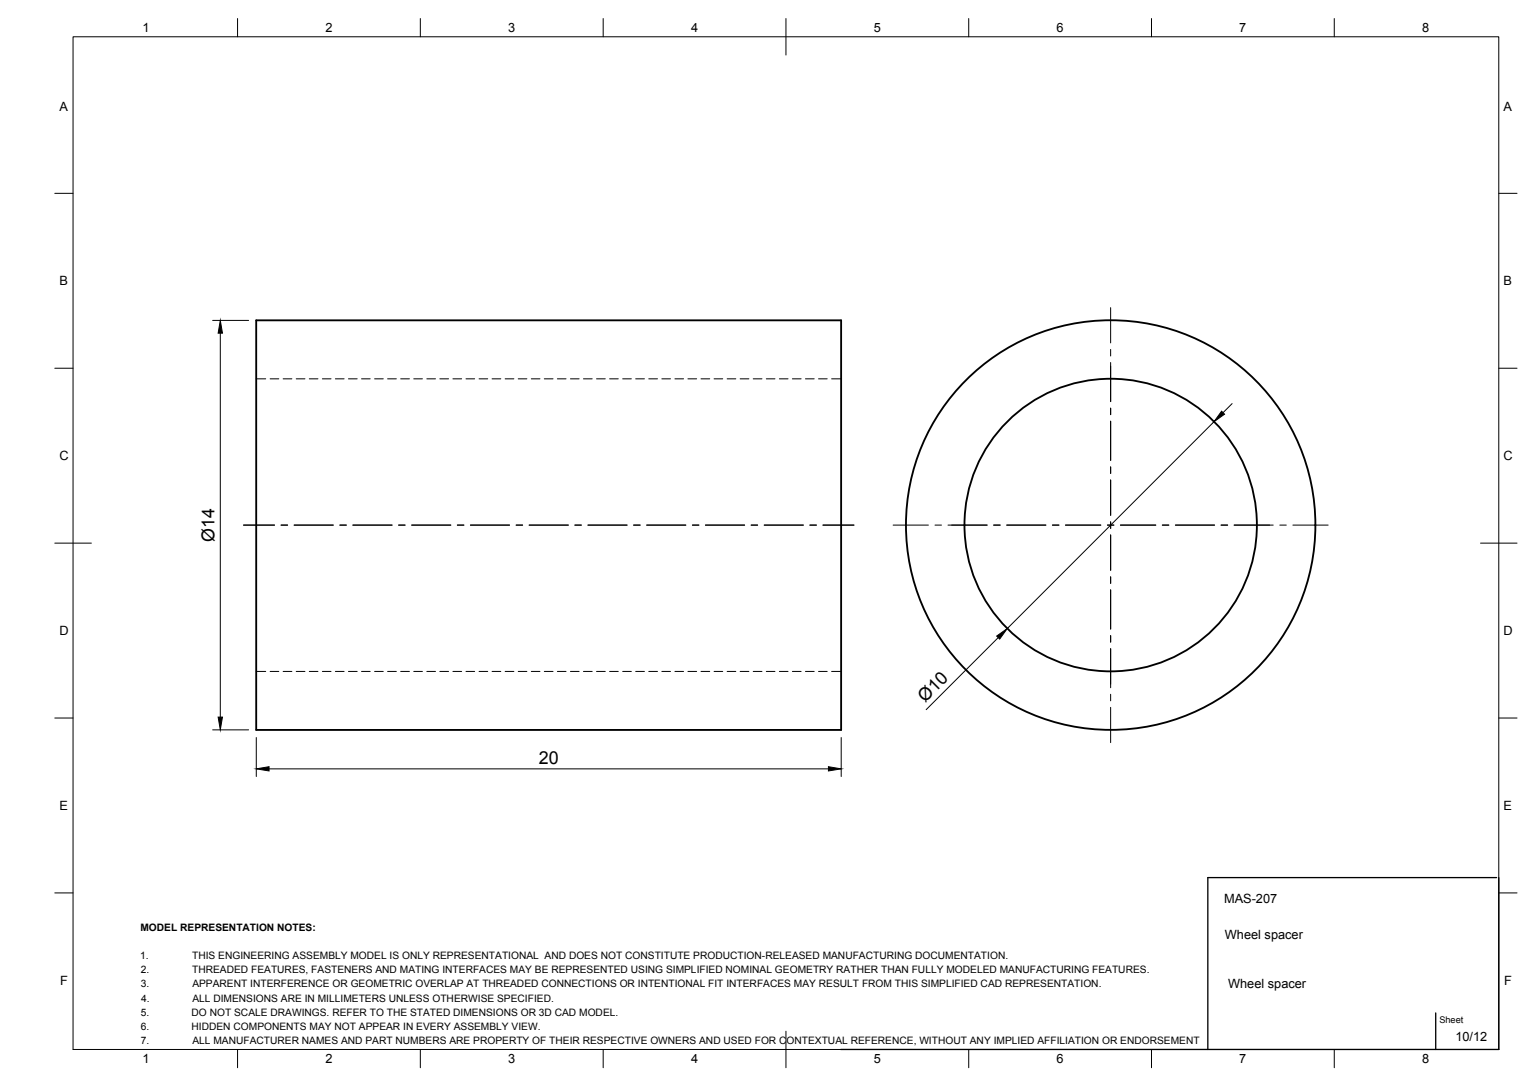
ISO-10303-21;
HEADER;
/* Generated by software containing ST-Developer
 * from STEP Tools, Inc. (www.steptools.com) 
 */

FILE_DESCRIPTION(
/* description */ ('Independent six-slot Geneva indexer. Center distance100, drive radius
50, 60degree indexing per input revolution with120degree engagement an
d240degree dwell. Native machined concave locking faces and relieved d
isk; replaceable retained drive pin; keyed output shaft. Geometry traj
ectory checks use calculated indexing positions, not a contact-dynamic
s simulation. No load or production rating assigned.'),
/* implementation_level */ '2;1');

FILE_NAME(
/* name */ 'Wheel spacer.step',
/* time_stamp */ '2026-11-09T17:53:22-08:00',
/* author */ (''),
/* organization */ (''),
/* preprocessor_version */ 'ST-DEVELOPER v20.2',
/* originating_system */ 'Autodesk Translation Framework v15.17.0.0',
/* authorisation */ '');

FILE_SCHEMA (('AUTOMOTIVE_DESIGN { 1 0 10303 214 3 1 1 }'));
ENDSEC;

DATA;
#10=MECHANICAL_DESIGN_GEOMETRIC_PRESENTATION_REPRESENTATION('',(#108),#4149);
#86=SHAPE_REPRESENTATION_RELATIONSHIP('SRR','None',#4203,#97);
#97=ADVANCED_BREP_SHAPE_REPRESENTATION('',(#119),#4145);
#108=STYLED_ITEM('',(#4266),#119);
#119=MANIFOLD_SOLID_BREP('Body1',#2302);
#155=FACE_BOUND('',#527,.T.);
#156=FACE_BOUND('',#529,.T.);
#228=PLANE('',#2669);
#229=PLANE('',#2670);
#356=FACE_OUTER_BOUND('',#524,.T.);
#357=FACE_OUTER_BOUND('',#525,.T.);
#358=FACE_OUTER_BOUND('',#526,.T.);
#359=FACE_OUTER_BOUND('',#528,.T.);
#524=EDGE_LOOP('',(#2040,#2041,#2042,#2043));
#525=EDGE_LOOP('',(#2044,#2045,#2046,#2047));
#526=EDGE_LOOP('',(#2048));
#527=EDGE_LOOP('',(#2049));
#528=EDGE_LOOP('',(#2050));
#529=EDGE_LOOP('',(#2051));
#706=LINE('',#4040,#878);
#707=LINE('',#4046,#879);
#878=VECTOR('',#3349,5.);
#879=VECTOR('',#3356,7.);
#1000=CIRCLE('',#2664,5.);
#1001=CIRCLE('',#2665,5.);
#1002=CIRCLE('',#2667,7.);
#1003=CIRCLE('',#2668,7.);
#1192=VERTEX_POINT('',#4037);
#1193=VERTEX_POINT('',#4039);
#1194=VERTEX_POINT('',#4043);
#1195=VERTEX_POINT('',#4045);
#1478=EDGE_CURVE('',#1192,#1192,#1000,.T.);
#1479=EDGE_CURVE('',#1192,#1193,#706,.T.);
#1480=EDGE_CURVE('',#1193,#1193,#1001,.T.);
#1481=EDGE_CURVE('',#1194,#1194,#1002,.T.);
#1482=EDGE_CURVE('',#1194,#1195,#707,.T.);
#1483=EDGE_CURVE('',#1195,#1195,#1003,.T.);
#2040=ORIENTED_EDGE('',*,*,#1478,.F.);
#2041=ORIENTED_EDGE('',*,*,#1479,.T.);
#2042=ORIENTED_EDGE('',*,*,#1480,.T.);
#2043=ORIENTED_EDGE('',*,*,#1479,.F.);
#2044=ORIENTED_EDGE('',*,*,#1481,.F.);
#2045=ORIENTED_EDGE('',*,*,#1482,.T.);
#2046=ORIENTED_EDGE('',*,*,#1483,.T.);
#2047=ORIENTED_EDGE('',*,*,#1482,.F.);
#2048=ORIENTED_EDGE('',*,*,#1481,.T.);
#2049=ORIENTED_EDGE('',*,*,#1478,.T.);
#2050=ORIENTED_EDGE('',*,*,#1483,.F.);
#2051=ORIENTED_EDGE('',*,*,#1480,.F.);
#2151=CYLINDRICAL_SURFACE('',#2663,5.);
#2152=CYLINDRICAL_SURFACE('',#2666,7.);
#2277=ADVANCED_FACE('',(#356),#2151,.F.);
#2278=ADVANCED_FACE('',(#357),#2152,.T.);
#2279=ADVANCED_FACE('',(#358,#155),#228,.T.);
#2280=ADVANCED_FACE('',(#359,#156),#229,.F.);
#2302=CLOSED_SHELL('',(#2277,#2278,#2279,#2280));
#2662=AXIS2_PLACEMENT_3D('',#4035,#3343,#3344);
#2663=AXIS2_PLACEMENT_3D('',#4036,#3345,#3346);
#2664=AXIS2_PLACEMENT_3D('',#4038,#3347,#3348);
#2665=AXIS2_PLACEMENT_3D('',#4041,#3350,#3351);
#2666=AXIS2_PLACEMENT_3D('',#4042,#3352,#3353);
#2667=AXIS2_PLACEMENT_3D('',#4044,#3354,#3355);
#2668=AXIS2_PLACEMENT_3D('',#4047,#3357,#3358);
#2669=AXIS2_PLACEMENT_3D('',#4048,#3359,#3360);
#2670=AXIS2_PLACEMENT_3D('',#4049,#3361,#3362);
#3343=DIRECTION('axis',(0.,0.,1.));
#3344=DIRECTION('refdir',(1.,0.,0.));
#3345=DIRECTION('center_axis',(0.,0.,1.));
#3346=DIRECTION('ref_axis',(1.,0.,0.));
#3347=DIRECTION('center_axis',(0.,0.,-1.));
#3348=DIRECTION('ref_axis',(1.,0.,0.));
#3349=DIRECTION('',(0.,0.,-1.));
#3350=DIRECTION('center_axis',(0.,0.,-1.));
#3351=DIRECTION('ref_axis',(1.,0.,0.));
#3352=DIRECTION('center_axis',(0.,0.,1.));
#3353=DIRECTION('ref_axis',(1.,0.,0.));
#3354=DIRECTION('center_axis',(0.,0.,1.));
#3355=DIRECTION('ref_axis',(1.,0.,0.));
#3356=DIRECTION('',(0.,0.,-1.));
#3357=DIRECTION('center_axis',(0.,0.,1.));
#3358=DIRECTION('ref_axis',(1.,0.,0.));
#3359=DIRECTION('center_axis',(0.,0.,1.));
#3360=DIRECTION('ref_axis',(1.,0.,0.));
#3361=DIRECTION('center_axis',(0.,0.,1.));
#3362=DIRECTION('ref_axis',(1.,0.,0.));
#4035=CARTESIAN_POINT('',(0.,0.,0.));
#4036=CARTESIAN_POINT('Origin',(0.,0.,0.));
#4037=CARTESIAN_POINT('',(-5.,-6.12323399573677E-16,20.));
#4038=CARTESIAN_POINT('Origin',(0.,0.,20.));
#4039=CARTESIAN_POINT('',(-5.,-6.12323399573677E-16,0.));
#4040=CARTESIAN_POINT('',(-5.,-6.12323399573677E-16,0.));
#4041=CARTESIAN_POINT('Origin',(0.,0.,0.));
#4042=CARTESIAN_POINT('Origin',(0.,0.,0.));
#4043=CARTESIAN_POINT('',(-7.,-8.57252759403147E-16,20.));
#4044=CARTESIAN_POINT('Origin',(0.,0.,20.));
#4045=CARTESIAN_POINT('',(-7.,-8.57252759403147E-16,0.));
#4046=CARTESIAN_POINT('',(-7.,-8.57252759403147E-16,0.));
#4047=CARTESIAN_POINT('Origin',(0.,0.,0.));
#4048=CARTESIAN_POINT('Origin',(0.,0.,20.));
#4049=CARTESIAN_POINT('Origin',(0.,0.,0.));
#4132=UNCERTAINTY_MEASURE_WITH_UNIT(LENGTH_MEASURE(0.01),#4150,
'DISTANCE_ACCURACY_VALUE',
'Maximum model space distance between geometric entities at asserted c
onnectivities');
#4136=UNCERTAINTY_MEASURE_WITH_UNIT(LENGTH_MEASURE(0.01),#4150,
'DISTANCE_ACCURACY_VALUE',
'Maximum model space distance between geometric entities at asserted c
onnectivities');
#4145=(
GEOMETRIC_REPRESENTATION_CONTEXT(3)
GLOBAL_UNCERTAINTY_ASSIGNED_CONTEXT((#4132))
GLOBAL_UNIT_ASSIGNED_CONTEXT((#4150,#4152,#4153))
REPRESENTATION_CONTEXT('','3D')
);
#4149=(
GEOMETRIC_REPRESENTATION_CONTEXT(3)
GLOBAL_UNCERTAINTY_ASSIGNED_CONTEXT((#4136))
GLOBAL_UNIT_ASSIGNED_CONTEXT((#4150,#4152,#4153))
REPRESENTATION_CONTEXT('','3D')
);
#4150=(
LENGTH_UNIT()
NAMED_UNIT(*)
SI_UNIT(.MILLI.,.METRE.)
);
#4152=(
NAMED_UNIT(*)
PLANE_ANGLE_UNIT()
SI_UNIT($,.RADIAN.)
);
#4153=(
NAMED_UNIT(*)
SI_UNIT($,.STERADIAN.)
SOLID_ANGLE_UNIT()
);
#4162=SHAPE_DEFINITION_REPRESENTATION(#4174,#4203);
#4174=PRODUCT_DEFINITION_SHAPE('',$,#4216);
#4203=SHAPE_REPRESENTATION('',(#2662),#4145);
#4207=PRODUCT_DEFINITION_CONTEXT('part definition',#4245,'design');
#4216=PRODUCT_DEFINITION('Wheel spacer','Wheel spacer',#4228,#4207);
#4228=PRODUCT_DEFINITION_FORMATION('',$,#4255);
#4245=APPLICATION_CONTEXT(
'Core Data for Automotive Mechanical Design Process');
#4246=PRODUCT_CONTEXT('part definition',#4245,'mechanical');
#4255=PRODUCT('Wheel spacer','Wheel spacer',$,(#4246));
#4266=PRESENTATION_STYLE_ASSIGNMENT((#4276));
#4276=SURFACE_STYLE_USAGE(.BOTH.,#4286);
#4286=SURFACE_SIDE_STYLE('',(#4296));
#4296=SURFACE_STYLE_FILL_AREA(#4306);
#4306=FILL_AREA_STYLE('Spacer gray',(#4316));
#4316=FILL_AREA_STYLE_COLOUR('Spacer gray',#4326);
#4326=COLOUR_RGB('Spacer gray',0.407843137254902,0.447058823529412,0.498039215686275);
ENDSEC;
END-ISO-10303-21;
